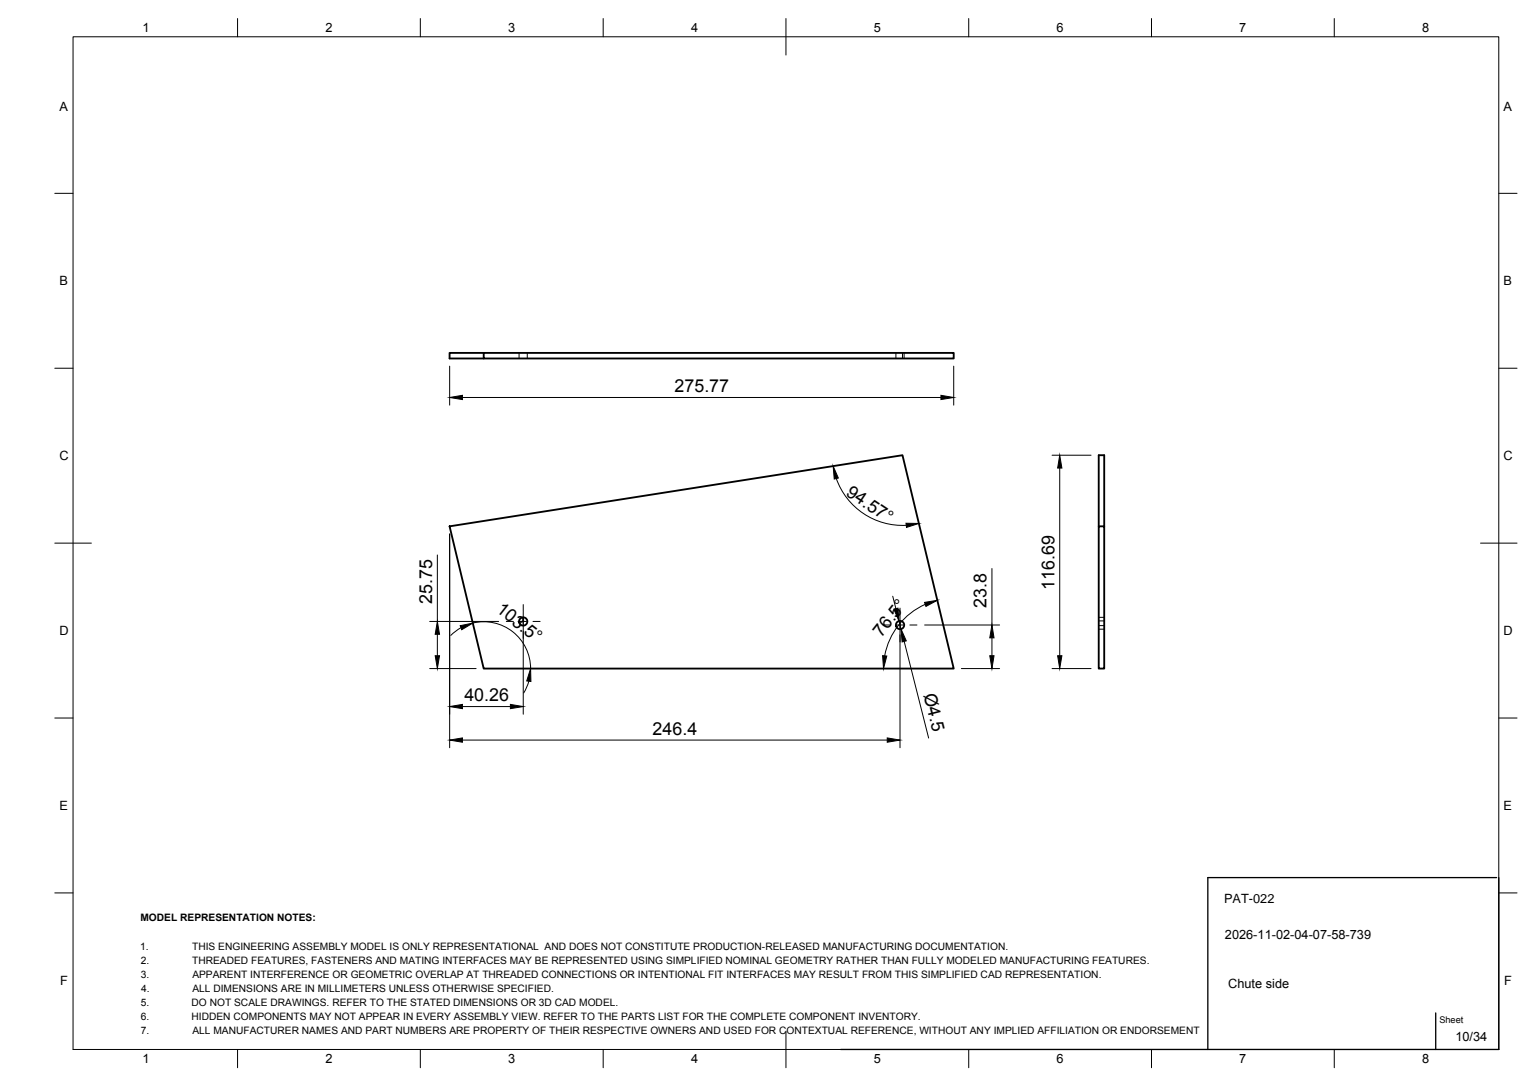
ISO-10303-21;
HEADER;
/* Generated by software containing ST-Developer
 * from STEP Tools, Inc. (www.steptools.com) 
 */

FILE_DESCRIPTION(
/* description */ ('Chute with adjustable gate'),
/* implementation_level */ '2;1');

FILE_NAME(
/* name */ 'Chute side.step',
/* time_stamp */ '2026-10-27T10:52:28-07:00',
/* author */ (''),
/* organization */ (''),
/* preprocessor_version */ 'ST-DEVELOPER v20.2',
/* originating_system */ 'Autodesk Translation Framework v15.17.0.0',
/* authorisation */ '');

FILE_SCHEMA (('AUTOMOTIVE_DESIGN { 1 0 10303 214 3 1 1 }'));
ENDSEC;

DATA;
#10=MECHANICAL_DESIGN_GEOMETRIC_PRESENTATION_REPRESENTATION('',(#419),#13094);
#355=SHAPE_REPRESENTATION_RELATIONSHIP('SRR','None',#13256,#387);
#387=ADVANCED_BREP_SHAPE_REPRESENTATION('',(#451),#13065);
#419=STYLED_ITEM('',(#13509),#451);
#451=MANIFOLD_SOLID_BREP('Body1',#7602);
#492=FACE_BOUND('',#1396,.T.);
#493=FACE_BOUND('',#1397,.T.);
#494=FACE_BOUND('',#1399,.T.);
#495=FACE_BOUND('',#1400,.T.);
#624=PLANE('',#8058);
#625=PLANE('',#8059);
#626=PLANE('',#8060);
#627=PLANE('',#8061);
#628=PLANE('',#8062);
#629=PLANE('',#8063);
#956=FACE_OUTER_BOUND('',#1389,.T.);
#957=FACE_OUTER_BOUND('',#1390,.T.);
#958=FACE_OUTER_BOUND('',#1391,.T.);
#959=FACE_OUTER_BOUND('',#1392,.T.);
#960=FACE_OUTER_BOUND('',#1393,.T.);
#961=FACE_OUTER_BOUND('',#1394,.T.);
#962=FACE_OUTER_BOUND('',#1395,.T.);
#963=FACE_OUTER_BOUND('',#1398,.T.);
#1389=EDGE_LOOP('',(#5378,#5379,#5380,#5381));
#1390=EDGE_LOOP('',(#5382,#5383,#5384,#5385));
#1391=EDGE_LOOP('',(#5386,#5387,#5388,#5389));
#1392=EDGE_LOOP('',(#5390,#5391,#5392,#5393));
#1393=EDGE_LOOP('',(#5394,#5395,#5396,#5397));
#1394=EDGE_LOOP('',(#5398,#5399,#5400,#5401));
#1395=EDGE_LOOP('',(#5402,#5403,#5404,#5405));
#1396=EDGE_LOOP('',(#5406));
#1397=EDGE_LOOP('',(#5407));
#1398=EDGE_LOOP('',(#5408,#5409,#5410,#5411));
#1399=EDGE_LOOP('',(#5412));
#1400=EDGE_LOOP('',(#5413));
#1940=LINE('',#11113,#2717);
#1941=LINE('',#11119,#2718);
#1942=LINE('',#11124,#2719);
#1943=LINE('',#11126,#2720);
#1944=LINE('',#11128,#2721);
#1945=LINE('',#11129,#2722);
#1946=LINE('',#11132,#2723);
#1947=LINE('',#11134,#2724);
#1948=LINE('',#11135,#2725);
#1949=LINE('',#11138,#2726);
#1950=LINE('',#11140,#2727);
#1951=LINE('',#11141,#2728);
#1952=LINE('',#11143,#2729);
#1953=LINE('',#11144,#2730);
#2717=VECTOR('',#8914,0.225);
#2718=VECTOR('',#8921,0.225000000000001);
#2719=VECTOR('',#8926,1.);
#2720=VECTOR('',#8927,1.);
#2721=VECTOR('',#8928,1.);
#2722=VECTOR('',#8929,1.);
#2723=VECTOR('',#8932,1.);
#2724=VECTOR('',#8933,1.);
#2725=VECTOR('',#8934,1.);
#2726=VECTOR('',#8937,1.);
#2727=VECTOR('',#8938,1.);
#2728=VECTOR('',#8939,1.);
#2729=VECTOR('',#8942,1.);
#2730=VECTOR('',#8943,1.);
#3430=CIRCLE('',#8053,0.225);
#3431=CIRCLE('',#8054,0.225);
#3432=CIRCLE('',#8056,0.225000000000001);
#3433=CIRCLE('',#8057,0.225000000000001);
#3657=VERTEX_POINT('',#11110);
#3658=VERTEX_POINT('',#11112);
#3659=VERTEX_POINT('',#11116);
#3660=VERTEX_POINT('',#11118);
#3661=VERTEX_POINT('',#11122);
#3662=VERTEX_POINT('',#11123);
#3663=VERTEX_POINT('',#11125);
#3664=VERTEX_POINT('',#11127);
#3665=VERTEX_POINT('',#11131);
#3666=VERTEX_POINT('',#11133);
#3667=VERTEX_POINT('',#11137);
#3668=VERTEX_POINT('',#11139);
#4322=EDGE_CURVE('',#3657,#3657,#3430,.T.);
#4323=EDGE_CURVE('',#3657,#3658,#1940,.T.);
#4324=EDGE_CURVE('',#3658,#3658,#3431,.T.);
#4325=EDGE_CURVE('',#3659,#3659,#3432,.T.);
#4326=EDGE_CURVE('',#3659,#3660,#1941,.T.);
#4327=EDGE_CURVE('',#3660,#3660,#3433,.T.);
#4328=EDGE_CURVE('',#3661,#3662,#1942,.T.);
#4329=EDGE_CURVE('',#3661,#3663,#1943,.T.);
#4330=EDGE_CURVE('',#3664,#3663,#1944,.T.);
#4331=EDGE_CURVE('',#3662,#3664,#1945,.T.);
#4332=EDGE_CURVE('',#3662,#3665,#1946,.T.);
#4333=EDGE_CURVE('',#3666,#3664,#1947,.T.);
#4334=EDGE_CURVE('',#3665,#3666,#1948,.T.);
#4335=EDGE_CURVE('',#3665,#3667,#1949,.T.);
#4336=EDGE_CURVE('',#3668,#3666,#1950,.T.);
#4337=EDGE_CURVE('',#3667,#3668,#1951,.T.);
#4338=EDGE_CURVE('',#3667,#3661,#1952,.T.);
#4339=EDGE_CURVE('',#3663,#3668,#1953,.T.);
#5378=ORIENTED_EDGE('',*,*,#4322,.F.);
#5379=ORIENTED_EDGE('',*,*,#4323,.T.);
#5380=ORIENTED_EDGE('',*,*,#4324,.F.);
#5381=ORIENTED_EDGE('',*,*,#4323,.F.);
#5382=ORIENTED_EDGE('',*,*,#4325,.F.);
#5383=ORIENTED_EDGE('',*,*,#4326,.T.);
#5384=ORIENTED_EDGE('',*,*,#4327,.F.);
#5385=ORIENTED_EDGE('',*,*,#4326,.F.);
#5386=ORIENTED_EDGE('',*,*,#4328,.F.);
#5387=ORIENTED_EDGE('',*,*,#4329,.T.);
#5388=ORIENTED_EDGE('',*,*,#4330,.F.);
#5389=ORIENTED_EDGE('',*,*,#4331,.F.);
#5390=ORIENTED_EDGE('',*,*,#4332,.F.);
#5391=ORIENTED_EDGE('',*,*,#4331,.T.);
#5392=ORIENTED_EDGE('',*,*,#4333,.F.);
#5393=ORIENTED_EDGE('',*,*,#4334,.F.);
#5394=ORIENTED_EDGE('',*,*,#4335,.F.);
#5395=ORIENTED_EDGE('',*,*,#4334,.T.);
#5396=ORIENTED_EDGE('',*,*,#4336,.F.);
#5397=ORIENTED_EDGE('',*,*,#4337,.F.);
#5398=ORIENTED_EDGE('',*,*,#4338,.F.);
#5399=ORIENTED_EDGE('',*,*,#4337,.T.);
#5400=ORIENTED_EDGE('',*,*,#4339,.F.);
#5401=ORIENTED_EDGE('',*,*,#4329,.F.);
#5402=ORIENTED_EDGE('',*,*,#4339,.T.);
#5403=ORIENTED_EDGE('',*,*,#4336,.T.);
#5404=ORIENTED_EDGE('',*,*,#4333,.T.);
#5405=ORIENTED_EDGE('',*,*,#4330,.T.);
#5406=ORIENTED_EDGE('',*,*,#4324,.T.);
#5407=ORIENTED_EDGE('',*,*,#4327,.T.);
#5408=ORIENTED_EDGE('',*,*,#4338,.T.);
#5409=ORIENTED_EDGE('',*,*,#4328,.T.);
#5410=ORIENTED_EDGE('',*,*,#4332,.T.);
#5411=ORIENTED_EDGE('',*,*,#4335,.T.);
#5412=ORIENTED_EDGE('',*,*,#4322,.T.);
#5413=ORIENTED_EDGE('',*,*,#4325,.T.);
#7114=CYLINDRICAL_SURFACE('',#8052,0.225);
#7115=CYLINDRICAL_SURFACE('',#8055,0.225000000000001);
#7224=ADVANCED_FACE('',(#956),#7114,.F.);
#7225=ADVANCED_FACE('',(#957),#7115,.F.);
#7226=ADVANCED_FACE('',(#958),#624,.T.);
#7227=ADVANCED_FACE('',(#959),#625,.T.);
#7228=ADVANCED_FACE('',(#960),#626,.T.);
#7229=ADVANCED_FACE('',(#961),#627,.T.);
#7230=ADVANCED_FACE('',(#962,#492,#493),#628,.T.);
#7231=ADVANCED_FACE('',(#963,#494,#495),#629,.F.);
#7602=CLOSED_SHELL('',(#7224,#7225,#7226,#7227,#7228,#7229,#7230,#7231));
#8051=AXIS2_PLACEMENT_3D('',#11108,#8908,#8909);
#8052=AXIS2_PLACEMENT_3D('',#11109,#8910,#8911);
#8053=AXIS2_PLACEMENT_3D('',#11111,#8912,#8913);
#8054=AXIS2_PLACEMENT_3D('',#11114,#8915,#8916);
#8055=AXIS2_PLACEMENT_3D('',#11115,#8917,#8918);
#8056=AXIS2_PLACEMENT_3D('',#11117,#8919,#8920);
#8057=AXIS2_PLACEMENT_3D('',#11120,#8922,#8923);
#8058=AXIS2_PLACEMENT_3D('',#11121,#8924,#8925);
#8059=AXIS2_PLACEMENT_3D('',#11130,#8930,#8931);
#8060=AXIS2_PLACEMENT_3D('',#11136,#8935,#8936);
#8061=AXIS2_PLACEMENT_3D('',#11142,#8940,#8941);
#8062=AXIS2_PLACEMENT_3D('',#11145,#8944,#8945);
#8063=AXIS2_PLACEMENT_3D('',#11146,#8946,#8947);
#8908=DIRECTION('axis',(0.,0.,1.));
#8909=DIRECTION('refdir',(1.,0.,0.));
#8910=DIRECTION('center_axis',(0.,1.,0.));
#8911=DIRECTION('ref_axis',(1.,0.,0.));
#8912=DIRECTION('center_axis',(0.,1.,0.));
#8913=DIRECTION('ref_axis',(1.,0.,0.));
#8914=DIRECTION('',(0.,1.,0.));
#8915=DIRECTION('center_axis',(0.,-1.,0.));
#8916=DIRECTION('ref_axis',(1.,0.,0.));
#8917=DIRECTION('center_axis',(0.,1.,0.));
#8918=DIRECTION('ref_axis',(1.,0.,0.));
#8919=DIRECTION('center_axis',(0.,1.,0.));
#8920=DIRECTION('ref_axis',(1.,0.,0.));
#8921=DIRECTION('',(0.,1.,0.));
#8922=DIRECTION('center_axis',(0.,-1.,0.));
#8923=DIRECTION('ref_axis',(1.,0.,0.));
#8924=DIRECTION('center_axis',(-1.,0.,0.));
#8925=DIRECTION('ref_axis',(0.,0.,1.));
#8926=DIRECTION('',(0.,0.,-1.));
#8927=DIRECTION('',(0.,1.,0.));
#8928=DIRECTION('',(0.,0.,1.));
#8929=DIRECTION('',(0.,1.,0.));
#8930=DIRECTION('center_axis',(0.233372952475324,0.,-0.972387301980517));
#8931=DIRECTION('ref_axis',(-0.972387301980517,0.,-0.233372952475324));
#8932=DIRECTION('',(0.972387301980517,0.,0.233372952475324));
#8933=DIRECTION('',(-0.972387301980517,0.,-0.233372952475324));
#8934=DIRECTION('',(0.,1.,0.));
#8935=DIRECTION('center_axis',(1.,0.,0.));
#8936=DIRECTION('ref_axis',(0.,0.,-1.));
#8937=DIRECTION('',(0.,0.,1.));
#8938=DIRECTION('',(0.,0.,-1.));
#8939=DIRECTION('',(0.,1.,0.));
#8940=DIRECTION('center_axis',(-0.07974522228289,0.,0.996815278536125));
#8941=DIRECTION('ref_axis',(0.996815278536125,0.,0.07974522228289));
#8942=DIRECTION('',(-0.996815278536125,0.,-0.07974522228289));
#8943=DIRECTION('',(0.996815278536125,0.,0.07974522228289));
#8944=DIRECTION('center_axis',(0.,1.,0.));
#8945=DIRECTION('ref_axis',(0.,0.,1.));
#8946=DIRECTION('center_axis',(0.,1.,0.));
#8947=DIRECTION('ref_axis',(1.,0.,0.));
#11108=CARTESIAN_POINT('',(0.,0.,0.));
#11109=CARTESIAN_POINT('Origin',(2.3,-7.9,7.));
#11110=CARTESIAN_POINT('',(2.075,-7.8,7.));
#11111=CARTESIAN_POINT('Origin',(2.3,-7.8,7.));
#11112=CARTESIAN_POINT('',(2.075,-7.5,7.));
#11113=CARTESIAN_POINT('',(2.075,-7.9,7.));
#11114=CARTESIAN_POINT('Origin',(2.3,-7.5,7.));
#11115=CARTESIAN_POINT('Origin',(22.3,-7.9,12.));
#11116=CARTESIAN_POINT('',(22.075,-7.8,12.));
#11117=CARTESIAN_POINT('Origin',(22.3,-7.8,12.));
#11118=CARTESIAN_POINT('',(22.075,-7.5,12.));
#11119=CARTESIAN_POINT('',(22.075,-7.9,12.));
#11120=CARTESIAN_POINT('Origin',(22.3,-7.5,12.));
#11121=CARTESIAN_POINT('Origin',(0.,-7.8,4.));
#11122=CARTESIAN_POINT('',(0.,-7.8,16.));
#11123=CARTESIAN_POINT('',(0.,-7.8,4.));
#11124=CARTESIAN_POINT('',(0.,-7.8,16.));
#11125=CARTESIAN_POINT('',(0.,-7.5,16.));
#11126=CARTESIAN_POINT('',(0.,-7.8,16.));
#11127=CARTESIAN_POINT('',(0.,-7.5,4.));
#11128=CARTESIAN_POINT('',(0.,-7.5,16.));
#11129=CARTESIAN_POINT('',(0.,-7.8,4.));
#11130=CARTESIAN_POINT('Origin',(25.,-7.8,10.));
#11131=CARTESIAN_POINT('',(25.,-7.8,10.));
#11132=CARTESIAN_POINT('',(0.,-7.8,4.));
#11133=CARTESIAN_POINT('',(25.,-7.5,10.));
#11134=CARTESIAN_POINT('',(0.,-7.5,4.));
#11135=CARTESIAN_POINT('',(25.,-7.8,10.));
#11136=CARTESIAN_POINT('Origin',(25.,-7.8,18.));
#11137=CARTESIAN_POINT('',(25.,-7.8,18.));
#11138=CARTESIAN_POINT('',(25.,-7.8,10.));
#11139=CARTESIAN_POINT('',(25.,-7.5,18.));
#11140=CARTESIAN_POINT('',(25.,-7.5,10.));
#11141=CARTESIAN_POINT('',(25.,-7.8,18.));
#11142=CARTESIAN_POINT('Origin',(0.,-7.8,16.));
#11143=CARTESIAN_POINT('',(25.,-7.8,18.));
#11144=CARTESIAN_POINT('',(25.,-7.5,18.));
#11145=CARTESIAN_POINT('Origin',(12.5,-7.5,11.));
#11146=CARTESIAN_POINT('Origin',(12.5,-7.8,11.));
#13028=UNCERTAINTY_MEASURE_WITH_UNIT(LENGTH_MEASURE(0.001),#13095,
'DISTANCE_ACCURACY_VALUE',
'Maximum model space distance between geometric entities at asserted c
onnectivities');
#13057=UNCERTAINTY_MEASURE_WITH_UNIT(LENGTH_MEASURE(0.001),#13095,
'DISTANCE_ACCURACY_VALUE',
'Maximum model space distance between geometric entities at asserted c
onnectivities');
#13065=(
GEOMETRIC_REPRESENTATION_CONTEXT(3)
GLOBAL_UNCERTAINTY_ASSIGNED_CONTEXT((#13028))
GLOBAL_UNIT_ASSIGNED_CONTEXT((#13095,#13097,#13098))
REPRESENTATION_CONTEXT('','3D')
);
#13094=(
GEOMETRIC_REPRESENTATION_CONTEXT(3)
GLOBAL_UNCERTAINTY_ASSIGNED_CONTEXT((#13057))
GLOBAL_UNIT_ASSIGNED_CONTEXT((#13095,#13097,#13098))
REPRESENTATION_CONTEXT('','3D')
);
#13095=(
LENGTH_UNIT()
NAMED_UNIT(*)
SI_UNIT(.CENTI.,.METRE.)
);
#13097=(
NAMED_UNIT(*)
PLANE_ANGLE_UNIT()
SI_UNIT($,.RADIAN.)
);
#13098=(
NAMED_UNIT(*)
SI_UNIT($,.STERADIAN.)
SOLID_ANGLE_UNIT()
);
#13106=SHAPE_DEFINITION_REPRESENTATION(#13142,#13256);
#13142=PRODUCT_DEFINITION_SHAPE('',$,#13293);
#13256=SHAPE_REPRESENTATION('',(#8051),#13065);
#13285=PRODUCT_DEFINITION_CONTEXT('part definition',#13395,'design');
#13293=PRODUCT_DEFINITION('Chute side','Chute side',#13329,#13285);
#13329=PRODUCT_DEFINITION_FORMATION('',$,#13404);
#13395=APPLICATION_CONTEXT(
'Core Data for Automotive Mechanical Design Process');
#13396=PRODUCT_CONTEXT('part definition',#13395,'mechanical');
#13404=PRODUCT('Chute side','Chute side','Chute side',(#13396));
#13503=COLOUR_RGB('Off White',0.89,0.88,0.83);
#13504=FILL_AREA_STYLE_COLOUR('',#13503);
#13505=FILL_AREA_STYLE('',(#13504));
#13506=SURFACE_STYLE_FILL_AREA(#13505);
#13507=SURFACE_SIDE_STYLE('',(#13506));
#13508=SURFACE_STYLE_USAGE(.BOTH.,#13507);
#13509=PRESENTATION_STYLE_ASSIGNMENT((#13508));
ENDSEC;
END-ISO-10303-21;
